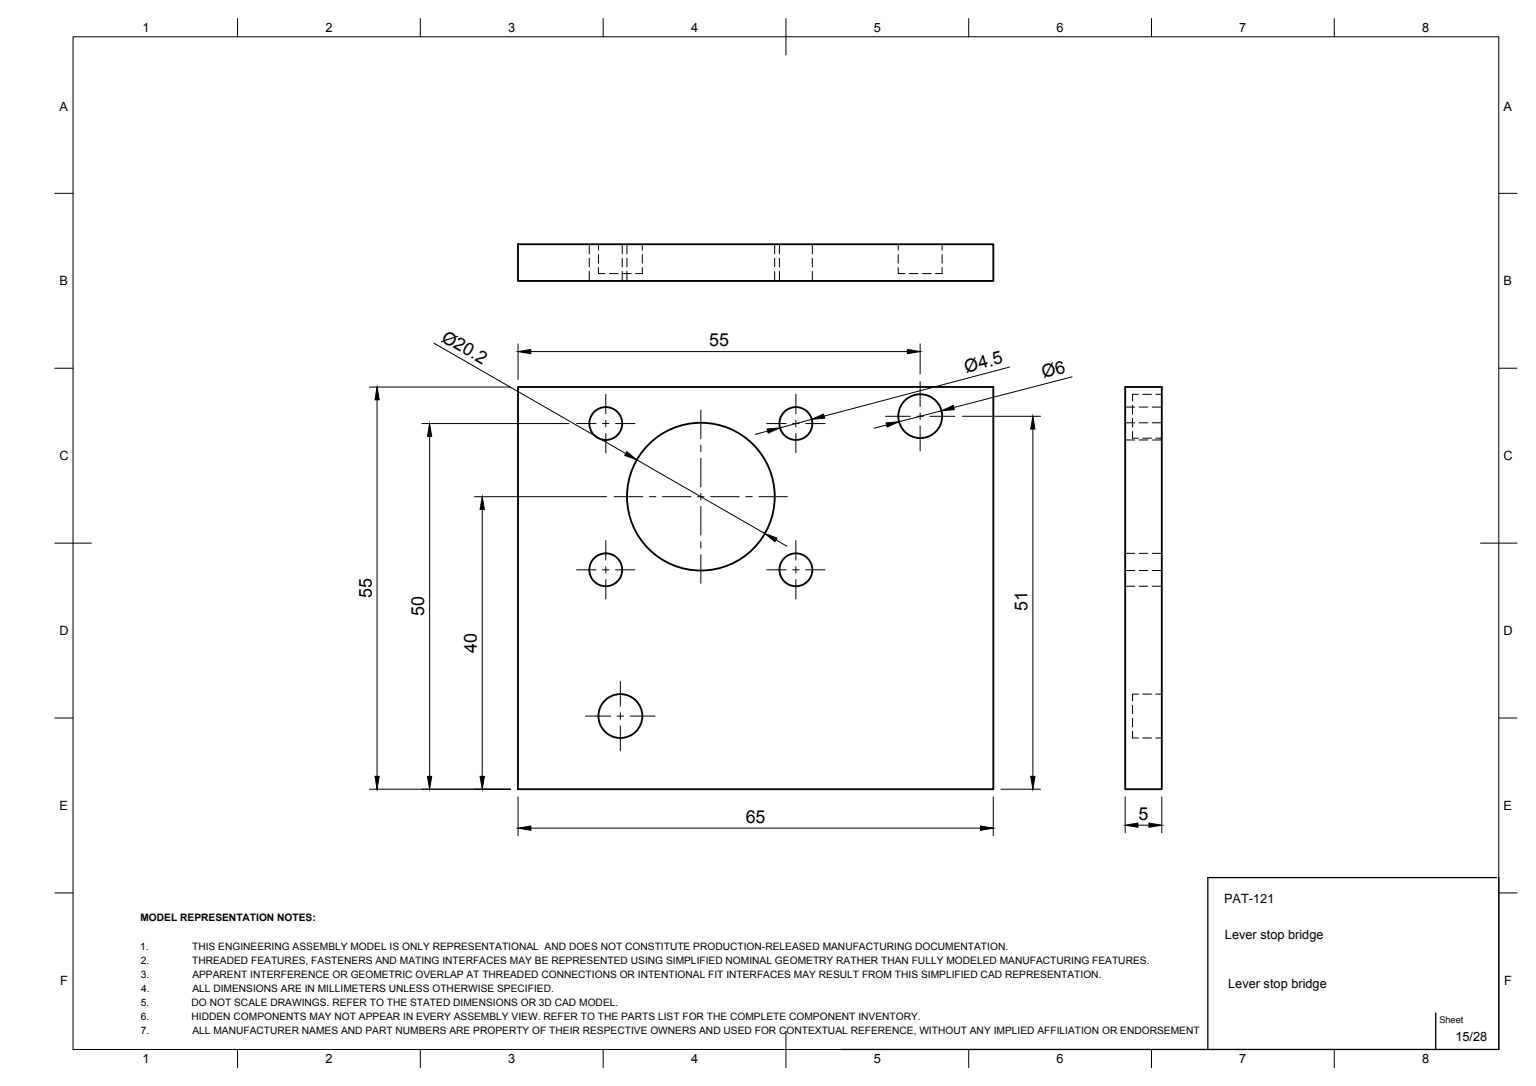
ISO-10303-21;
HEADER;
/* Generated by software containing ST-Developer
 * from STEP Tools, Inc. (www.steptools.com) 
 */

FILE_DESCRIPTION(
/* description */ ('Wall-mounted air drop station'),
/* implementation_level */ '2;1');

FILE_NAME(
/* name */ 'Lever stop bridge.step',
/* time_stamp */ '2026-10-28T22:16:19-07:00',
/* author */ (''),
/* organization */ (''),
/* preprocessor_version */ 'ST-DEVELOPER v20.2',
/* originating_system */ 'Autodesk Translation Framework v15.17.0.0',
/* authorisation */ '');

FILE_SCHEMA (('AUTOMOTIVE_DESIGN { 1 0 10303 214 3 1 1 }'));
ENDSEC;

DATA;
#10=MECHANICAL_DESIGN_GEOMETRIC_PRESENTATION_REPRESENTATION('',(#355),#10517);
#297=SHAPE_REPRESENTATION_RELATIONSHIP('SRR','None',#10654,#326);
#326=ADVANCED_BREP_SHAPE_REPRESENTATION('',(#384),#10498);
#355=STYLED_ITEM('',(#10860),#384);
#384=MANIFOLD_SOLID_BREP('Body1',#5894);
#477=FACE_BOUND('',#1356,.T.);
#478=FACE_BOUND('',#1357,.T.);
#479=FACE_BOUND('',#1358,.T.);
#480=FACE_BOUND('',#1359,.T.);
#481=FACE_BOUND('',#1360,.T.);
#482=FACE_BOUND('',#1361,.T.);
#483=FACE_BOUND('',#1362,.T.);
#484=FACE_BOUND('',#1364,.T.);
#485=FACE_BOUND('',#1365,.T.);
#486=FACE_BOUND('',#1366,.T.);
#487=FACE_BOUND('',#1367,.T.);
#488=FACE_BOUND('',#1368,.T.);
#619=PLANE('',#6528);
#620=PLANE('',#6532);
#621=PLANE('',#6548);
#622=PLANE('',#6549);
#623=PLANE('',#6550);
#624=PLANE('',#6551);
#625=PLANE('',#6552);
#626=PLANE('',#6553);
#909=FACE_OUTER_BOUND('',#1342,.T.);
#910=FACE_OUTER_BOUND('',#1343,.T.);
#911=FACE_OUTER_BOUND('',#1344,.T.);
#912=FACE_OUTER_BOUND('',#1345,.T.);
#913=FACE_OUTER_BOUND('',#1346,.T.);
#914=FACE_OUTER_BOUND('',#1347,.T.);
#915=FACE_OUTER_BOUND('',#1348,.T.);
#916=FACE_OUTER_BOUND('',#1349,.T.);
#917=FACE_OUTER_BOUND('',#1350,.T.);
#918=FACE_OUTER_BOUND('',#1351,.T.);
#919=FACE_OUTER_BOUND('',#1352,.T.);
#920=FACE_OUTER_BOUND('',#1353,.T.);
#921=FACE_OUTER_BOUND('',#1354,.T.);
#922=FACE_OUTER_BOUND('',#1355,.T.);
#923=FACE_OUTER_BOUND('',#1363,.T.);
#1342=EDGE_LOOP('',(#4631,#4632,#4633,#4634));
#1343=EDGE_LOOP('',(#4635));
#1344=EDGE_LOOP('',(#4636,#4637,#4638,#4639));
#1345=EDGE_LOOP('',(#4640));
#1346=EDGE_LOOP('',(#4641,#4642,#4643,#4644));
#1347=EDGE_LOOP('',(#4645,#4646,#4647,#4648));
#1348=EDGE_LOOP('',(#4649,#4650,#4651,#4652));
#1349=EDGE_LOOP('',(#4653,#4654,#4655,#4656));
#1350=EDGE_LOOP('',(#4657,#4658,#4659,#4660));
#1351=EDGE_LOOP('',(#4661,#4662,#4663,#4664));
#1352=EDGE_LOOP('',(#4665,#4666,#4667,#4668));
#1353=EDGE_LOOP('',(#4669,#4670,#4671,#4672));
#1354=EDGE_LOOP('',(#4673,#4674,#4675,#4676));
#1355=EDGE_LOOP('',(#4677,#4678,#4679,#4680));
#1356=EDGE_LOOP('',(#4681));
#1357=EDGE_LOOP('',(#4682));
#1358=EDGE_LOOP('',(#4683));
#1359=EDGE_LOOP('',(#4684));
#1360=EDGE_LOOP('',(#4685));
#1361=EDGE_LOOP('',(#4686));
#1362=EDGE_LOOP('',(#4687));
#1363=EDGE_LOOP('',(#4688,#4689,#4690,#4691));
#1364=EDGE_LOOP('',(#4692));
#1365=EDGE_LOOP('',(#4693));
#1366=EDGE_LOOP('',(#4694));
#1367=EDGE_LOOP('',(#4695));
#1368=EDGE_LOOP('',(#4696));
#1799=LINE('',#9486,#2263);
#1800=LINE('',#9493,#2264);
#1801=LINE('',#9500,#2265);
#1802=LINE('',#9506,#2266);
#1803=LINE('',#9512,#2267);
#1804=LINE('',#9518,#2268);
#1805=LINE('',#9524,#2269);
#1806=LINE('',#9529,#2270);
#1807=LINE('',#9531,#2271);
#1808=LINE('',#9533,#2272);
#1809=LINE('',#9534,#2273);
#1810=LINE('',#9537,#2274);
#1811=LINE('',#9539,#2275);
#1812=LINE('',#9540,#2276);
#1813=LINE('',#9543,#2277);
#1814=LINE('',#9545,#2278);
#1815=LINE('',#9546,#2279);
#1816=LINE('',#9548,#2280);
#1817=LINE('',#9549,#2281);
#2263=VECTOR('',#7715,0.3);
#2264=VECTOR('',#7724,0.3);
#2265=VECTOR('',#7733,0.225);
#2266=VECTOR('',#7740,0.225);
#2267=VECTOR('',#7747,0.225);
#2268=VECTOR('',#7754,0.225);
#2269=VECTOR('',#7761,1.01);
#2270=VECTOR('',#7766,1.);
#2271=VECTOR('',#7767,1.);
#2272=VECTOR('',#7768,1.);
#2273=VECTOR('',#7769,1.);
#2274=VECTOR('',#7772,1.);
#2275=VECTOR('',#7773,1.);
#2276=VECTOR('',#7774,1.);
#2277=VECTOR('',#7777,1.);
#2278=VECTOR('',#7778,1.);
#2279=VECTOR('',#7779,1.);
#2280=VECTOR('',#7782,1.);
#2281=VECTOR('',#7783,1.);
#2642=CIRCLE('',#6526,0.3);
#2643=CIRCLE('',#6527,0.3);
#2644=CIRCLE('',#6530,0.3);
#2645=CIRCLE('',#6531,0.3);
#2646=CIRCLE('',#6534,0.225);
#2647=CIRCLE('',#6535,0.225);
#2648=CIRCLE('',#6537,0.225);
#2649=CIRCLE('',#6538,0.225);
#2650=CIRCLE('',#6540,0.225);
#2651=CIRCLE('',#6541,0.225);
#2652=CIRCLE('',#6543,0.225);
#2653=CIRCLE('',#6544,0.225);
#2654=CIRCLE('',#6546,1.01);
#2655=CIRCLE('',#6547,1.01);
#2984=VERTEX_POINT('',#9483);
#2985=VERTEX_POINT('',#9485);
#2986=VERTEX_POINT('',#9490);
#2987=VERTEX_POINT('',#9492);
#2988=VERTEX_POINT('',#9497);
#2989=VERTEX_POINT('',#9499);
#2990=VERTEX_POINT('',#9503);
#2991=VERTEX_POINT('',#9505);
#2992=VERTEX_POINT('',#9509);
#2993=VERTEX_POINT('',#9511);
#2994=VERTEX_POINT('',#9515);
#2995=VERTEX_POINT('',#9517);
#2996=VERTEX_POINT('',#9521);
#2997=VERTEX_POINT('',#9523);
#2998=VERTEX_POINT('',#9527);
#2999=VERTEX_POINT('',#9528);
#3000=VERTEX_POINT('',#9530);
#3001=VERTEX_POINT('',#9532);
#3002=VERTEX_POINT('',#9536);
#3003=VERTEX_POINT('',#9538);
#3004=VERTEX_POINT('',#9542);
#3005=VERTEX_POINT('',#9544);
#3573=EDGE_CURVE('',#2984,#2984,#2642,.T.);
#3574=EDGE_CURVE('',#2984,#2985,#1799,.T.);
#3575=EDGE_CURVE('',#2985,#2985,#2643,.T.);
#3576=EDGE_CURVE('',#2986,#2986,#2644,.T.);
#3577=EDGE_CURVE('',#2986,#2987,#1800,.T.);
#3578=EDGE_CURVE('',#2987,#2987,#2645,.T.);
#3579=EDGE_CURVE('',#2988,#2988,#2646,.T.);
#3580=EDGE_CURVE('',#2988,#2989,#1801,.T.);
#3581=EDGE_CURVE('',#2989,#2989,#2647,.T.);
#3582=EDGE_CURVE('',#2990,#2990,#2648,.T.);
#3583=EDGE_CURVE('',#2990,#2991,#1802,.T.);
#3584=EDGE_CURVE('',#2991,#2991,#2649,.T.);
#3585=EDGE_CURVE('',#2992,#2992,#2650,.T.);
#3586=EDGE_CURVE('',#2992,#2993,#1803,.T.);
#3587=EDGE_CURVE('',#2993,#2993,#2651,.T.);
#3588=EDGE_CURVE('',#2994,#2994,#2652,.T.);
#3589=EDGE_CURVE('',#2994,#2995,#1804,.T.);
#3590=EDGE_CURVE('',#2995,#2995,#2653,.T.);
#3591=EDGE_CURVE('',#2996,#2996,#2654,.T.);
#3592=EDGE_CURVE('',#2996,#2997,#1805,.T.);
#3593=EDGE_CURVE('',#2997,#2997,#2655,.T.);
#3594=EDGE_CURVE('',#2998,#2999,#1806,.T.);
#3595=EDGE_CURVE('',#2999,#3000,#1807,.T.);
#3596=EDGE_CURVE('',#3001,#3000,#1808,.T.);
#3597=EDGE_CURVE('',#2998,#3001,#1809,.T.);
#3598=EDGE_CURVE('',#3002,#2998,#1810,.T.);
#3599=EDGE_CURVE('',#3003,#3001,#1811,.T.);
#3600=EDGE_CURVE('',#3002,#3003,#1812,.T.);
#3601=EDGE_CURVE('',#3004,#3002,#1813,.T.);
#3602=EDGE_CURVE('',#3005,#3003,#1814,.T.);
#3603=EDGE_CURVE('',#3004,#3005,#1815,.T.);
#3604=EDGE_CURVE('',#2999,#3004,#1816,.T.);
#3605=EDGE_CURVE('',#3000,#3005,#1817,.T.);
#4631=ORIENTED_EDGE('',*,*,#3573,.F.);
#4632=ORIENTED_EDGE('',*,*,#3574,.T.);
#4633=ORIENTED_EDGE('',*,*,#3575,.F.);
#4634=ORIENTED_EDGE('',*,*,#3574,.F.);
#4635=ORIENTED_EDGE('',*,*,#3573,.T.);
#4636=ORIENTED_EDGE('',*,*,#3576,.F.);
#4637=ORIENTED_EDGE('',*,*,#3577,.T.);
#4638=ORIENTED_EDGE('',*,*,#3578,.F.);
#4639=ORIENTED_EDGE('',*,*,#3577,.F.);
#4640=ORIENTED_EDGE('',*,*,#3576,.T.);
#4641=ORIENTED_EDGE('',*,*,#3579,.F.);
#4642=ORIENTED_EDGE('',*,*,#3580,.T.);
#4643=ORIENTED_EDGE('',*,*,#3581,.F.);
#4644=ORIENTED_EDGE('',*,*,#3580,.F.);
#4645=ORIENTED_EDGE('',*,*,#3582,.F.);
#4646=ORIENTED_EDGE('',*,*,#3583,.T.);
#4647=ORIENTED_EDGE('',*,*,#3584,.F.);
#4648=ORIENTED_EDGE('',*,*,#3583,.F.);
#4649=ORIENTED_EDGE('',*,*,#3585,.F.);
#4650=ORIENTED_EDGE('',*,*,#3586,.T.);
#4651=ORIENTED_EDGE('',*,*,#3587,.F.);
#4652=ORIENTED_EDGE('',*,*,#3586,.F.);
#4653=ORIENTED_EDGE('',*,*,#3588,.F.);
#4654=ORIENTED_EDGE('',*,*,#3589,.T.);
#4655=ORIENTED_EDGE('',*,*,#3590,.F.);
#4656=ORIENTED_EDGE('',*,*,#3589,.F.);
#4657=ORIENTED_EDGE('',*,*,#3591,.F.);
#4658=ORIENTED_EDGE('',*,*,#3592,.T.);
#4659=ORIENTED_EDGE('',*,*,#3593,.F.);
#4660=ORIENTED_EDGE('',*,*,#3592,.F.);
#4661=ORIENTED_EDGE('',*,*,#3594,.T.);
#4662=ORIENTED_EDGE('',*,*,#3595,.T.);
#4663=ORIENTED_EDGE('',*,*,#3596,.F.);
#4664=ORIENTED_EDGE('',*,*,#3597,.F.);
#4665=ORIENTED_EDGE('',*,*,#3598,.T.);
#4666=ORIENTED_EDGE('',*,*,#3597,.T.);
#4667=ORIENTED_EDGE('',*,*,#3599,.F.);
#4668=ORIENTED_EDGE('',*,*,#3600,.F.);
#4669=ORIENTED_EDGE('',*,*,#3601,.T.);
#4670=ORIENTED_EDGE('',*,*,#3600,.T.);
#4671=ORIENTED_EDGE('',*,*,#3602,.F.);
#4672=ORIENTED_EDGE('',*,*,#3603,.F.);
#4673=ORIENTED_EDGE('',*,*,#3604,.T.);
#4674=ORIENTED_EDGE('',*,*,#3603,.T.);
#4675=ORIENTED_EDGE('',*,*,#3605,.F.);
#4676=ORIENTED_EDGE('',*,*,#3595,.F.);
#4677=ORIENTED_EDGE('',*,*,#3605,.T.);
#4678=ORIENTED_EDGE('',*,*,#3602,.T.);
#4679=ORIENTED_EDGE('',*,*,#3599,.T.);
#4680=ORIENTED_EDGE('',*,*,#3596,.T.);
#4681=ORIENTED_EDGE('',*,*,#3575,.T.);
#4682=ORIENTED_EDGE('',*,*,#3578,.T.);
#4683=ORIENTED_EDGE('',*,*,#3593,.T.);
#4684=ORIENTED_EDGE('',*,*,#3590,.T.);
#4685=ORIENTED_EDGE('',*,*,#3587,.T.);
#4686=ORIENTED_EDGE('',*,*,#3584,.T.);
#4687=ORIENTED_EDGE('',*,*,#3581,.T.);
#4688=ORIENTED_EDGE('',*,*,#3604,.F.);
#4689=ORIENTED_EDGE('',*,*,#3594,.F.);
#4690=ORIENTED_EDGE('',*,*,#3598,.F.);
#4691=ORIENTED_EDGE('',*,*,#3601,.F.);
#4692=ORIENTED_EDGE('',*,*,#3591,.T.);
#4693=ORIENTED_EDGE('',*,*,#3588,.T.);
#4694=ORIENTED_EDGE('',*,*,#3585,.T.);
#4695=ORIENTED_EDGE('',*,*,#3582,.T.);
#4696=ORIENTED_EDGE('',*,*,#3579,.T.);
#5486=CYLINDRICAL_SURFACE('',#6525,0.3);
#5487=CYLINDRICAL_SURFACE('',#6529,0.3);
#5488=CYLINDRICAL_SURFACE('',#6533,0.225);
#5489=CYLINDRICAL_SURFACE('',#6536,0.225);
#5490=CYLINDRICAL_SURFACE('',#6539,0.225);
#5491=CYLINDRICAL_SURFACE('',#6542,0.225);
#5492=CYLINDRICAL_SURFACE('',#6545,1.01);
#5682=ADVANCED_FACE('',(#909),#5486,.F.);
#5683=ADVANCED_FACE('',(#910),#619,.T.);
#5684=ADVANCED_FACE('',(#911),#5487,.F.);
#5685=ADVANCED_FACE('',(#912),#620,.T.);
#5686=ADVANCED_FACE('',(#913),#5488,.F.);
#5687=ADVANCED_FACE('',(#914),#5489,.F.);
#5688=ADVANCED_FACE('',(#915),#5490,.F.);
#5689=ADVANCED_FACE('',(#916),#5491,.F.);
#5690=ADVANCED_FACE('',(#917),#5492,.F.);
#5691=ADVANCED_FACE('',(#918),#621,.T.);
#5692=ADVANCED_FACE('',(#919),#622,.T.);
#5693=ADVANCED_FACE('',(#920),#623,.T.);
#5694=ADVANCED_FACE('',(#921),#624,.T.);
#5695=ADVANCED_FACE('',(#922,#477,#478,#479,#480,#481,#482,#483),#625,.T.);
#5696=ADVANCED_FACE('',(#923,#484,#485,#486,#487,#488),#626,.F.);
#5894=CLOSED_SHELL('',(#5682,#5683,#5684,#5685,#5686,#5687,#5688,#5689,
#5690,#5691,#5692,#5693,#5694,#5695,#5696));
#6524=AXIS2_PLACEMENT_3D('',#9481,#7709,#7710);
#6525=AXIS2_PLACEMENT_3D('',#9482,#7711,#7712);
#6526=AXIS2_PLACEMENT_3D('',#9484,#7713,#7714);
#6527=AXIS2_PLACEMENT_3D('',#9487,#7716,#7717);
#6528=AXIS2_PLACEMENT_3D('',#9488,#7718,#7719);
#6529=AXIS2_PLACEMENT_3D('',#9489,#7720,#7721);
#6530=AXIS2_PLACEMENT_3D('',#9491,#7722,#7723);
#6531=AXIS2_PLACEMENT_3D('',#9494,#7725,#7726);
#6532=AXIS2_PLACEMENT_3D('',#9495,#7727,#7728);
#6533=AXIS2_PLACEMENT_3D('',#9496,#7729,#7730);
#6534=AXIS2_PLACEMENT_3D('',#9498,#7731,#7732);
#6535=AXIS2_PLACEMENT_3D('',#9501,#7734,#7735);
#6536=AXIS2_PLACEMENT_3D('',#9502,#7736,#7737);
#6537=AXIS2_PLACEMENT_3D('',#9504,#7738,#7739);
#6538=AXIS2_PLACEMENT_3D('',#9507,#7741,#7742);
#6539=AXIS2_PLACEMENT_3D('',#9508,#7743,#7744);
#6540=AXIS2_PLACEMENT_3D('',#9510,#7745,#7746);
#6541=AXIS2_PLACEMENT_3D('',#9513,#7748,#7749);
#6542=AXIS2_PLACEMENT_3D('',#9514,#7750,#7751);
#6543=AXIS2_PLACEMENT_3D('',#9516,#7752,#7753);
#6544=AXIS2_PLACEMENT_3D('',#9519,#7755,#7756);
#6545=AXIS2_PLACEMENT_3D('',#9520,#7757,#7758);
#6546=AXIS2_PLACEMENT_3D('',#9522,#7759,#7760);
#6547=AXIS2_PLACEMENT_3D('',#9525,#7762,#7763);
#6548=AXIS2_PLACEMENT_3D('',#9526,#7764,#7765);
#6549=AXIS2_PLACEMENT_3D('',#9535,#7770,#7771);
#6550=AXIS2_PLACEMENT_3D('',#9541,#7775,#7776);
#6551=AXIS2_PLACEMENT_3D('',#9547,#7780,#7781);
#6552=AXIS2_PLACEMENT_3D('',#9550,#7784,#7785);
#6553=AXIS2_PLACEMENT_3D('',#9551,#7786,#7787);
#7709=DIRECTION('axis',(0.,0.,1.));
#7710=DIRECTION('refdir',(1.,0.,0.));
#7711=DIRECTION('center_axis',(0.,0.,1.));
#7712=DIRECTION('ref_axis',(1.,0.,0.));
#7713=DIRECTION('center_axis',(0.,0.,1.));
#7714=DIRECTION('ref_axis',(1.,0.,0.));
#7715=DIRECTION('',(0.,0.,1.));
#7716=DIRECTION('center_axis',(0.,0.,-1.));
#7717=DIRECTION('ref_axis',(1.,0.,0.));
#7718=DIRECTION('center_axis',(0.,0.,1.));
#7719=DIRECTION('ref_axis',(1.,0.,0.));
#7720=DIRECTION('center_axis',(0.,0.,1.));
#7721=DIRECTION('ref_axis',(1.,0.,0.));
#7722=DIRECTION('center_axis',(0.,0.,1.));
#7723=DIRECTION('ref_axis',(1.,0.,0.));
#7724=DIRECTION('',(0.,0.,1.));
#7725=DIRECTION('center_axis',(0.,0.,-1.));
#7726=DIRECTION('ref_axis',(1.,0.,0.));
#7727=DIRECTION('center_axis',(0.,0.,1.));
#7728=DIRECTION('ref_axis',(1.,0.,0.));
#7729=DIRECTION('center_axis',(0.,0.,1.));
#7730=DIRECTION('ref_axis',(1.,0.,0.));
#7731=DIRECTION('center_axis',(0.,0.,1.));
#7732=DIRECTION('ref_axis',(1.,0.,0.));
#7733=DIRECTION('',(0.,0.,1.));
#7734=DIRECTION('center_axis',(0.,0.,-1.));
#7735=DIRECTION('ref_axis',(1.,0.,0.));
#7736=DIRECTION('center_axis',(0.,0.,1.));
#7737=DIRECTION('ref_axis',(1.,0.,0.));
#7738=DIRECTION('center_axis',(0.,0.,1.));
#7739=DIRECTION('ref_axis',(1.,0.,0.));
#7740=DIRECTION('',(0.,0.,1.));
#7741=DIRECTION('center_axis',(0.,0.,-1.));
#7742=DIRECTION('ref_axis',(1.,0.,0.));
#7743=DIRECTION('center_axis',(0.,0.,1.));
#7744=DIRECTION('ref_axis',(1.,0.,0.));
#7745=DIRECTION('center_axis',(0.,0.,1.));
#7746=DIRECTION('ref_axis',(1.,0.,0.));
#7747=DIRECTION('',(0.,0.,1.));
#7748=DIRECTION('center_axis',(0.,0.,-1.));
#7749=DIRECTION('ref_axis',(1.,0.,0.));
#7750=DIRECTION('center_axis',(0.,0.,1.));
#7751=DIRECTION('ref_axis',(1.,0.,0.));
#7752=DIRECTION('center_axis',(0.,0.,1.));
#7753=DIRECTION('ref_axis',(1.,0.,0.));
#7754=DIRECTION('',(0.,0.,1.));
#7755=DIRECTION('center_axis',(0.,0.,-1.));
#7756=DIRECTION('ref_axis',(1.,0.,0.));
#7757=DIRECTION('center_axis',(0.,0.,1.));
#7758=DIRECTION('ref_axis',(1.,0.,0.));
#7759=DIRECTION('center_axis',(0.,0.,1.));
#7760=DIRECTION('ref_axis',(1.,0.,0.));
#7761=DIRECTION('',(0.,0.,1.));
#7762=DIRECTION('center_axis',(0.,0.,-1.));
#7763=DIRECTION('ref_axis',(1.,0.,0.));
#7764=DIRECTION('center_axis',(0.,1.,0.));
#7765=DIRECTION('ref_axis',(-1.,0.,0.));
#7766=DIRECTION('',(-1.,0.,0.));
#7767=DIRECTION('',(0.,0.,1.));
#7768=DIRECTION('',(-1.,0.,0.));
#7769=DIRECTION('',(0.,0.,1.));
#7770=DIRECTION('center_axis',(1.,0.,0.));
#7771=DIRECTION('ref_axis',(0.,1.,0.));
#7772=DIRECTION('',(0.,1.,0.));
#7773=DIRECTION('',(0.,1.,0.));
#7774=DIRECTION('',(0.,0.,1.));
#7775=DIRECTION('center_axis',(0.,-1.,0.));
#7776=DIRECTION('ref_axis',(1.,0.,0.));
#7777=DIRECTION('',(1.,0.,0.));
#7778=DIRECTION('',(1.,0.,0.));
#7779=DIRECTION('',(0.,0.,1.));
#7780=DIRECTION('center_axis',(-1.,0.,0.));
#7781=DIRECTION('ref_axis',(0.,-1.,0.));
#7782=DIRECTION('',(0.,-1.,0.));
#7783=DIRECTION('',(0.,-1.,0.));
#7784=DIRECTION('center_axis',(0.,0.,1.));
#7785=DIRECTION('ref_axis',(1.,0.,0.));
#7786=DIRECTION('center_axis',(0.,0.,1.));
#7787=DIRECTION('ref_axis',(1.,0.,0.));
#9481=CARTESIAN_POINT('',(0.,0.,0.));
#9482=CARTESIAN_POINT('Origin',(-1.1,-3.,8.1));
#9483=CARTESIAN_POINT('',(-1.4,-3.,8.1));
#9484=CARTESIAN_POINT('Origin',(-1.1,-3.,8.1));
#9485=CARTESIAN_POINT('',(-1.4,-3.,8.5));
#9486=CARTESIAN_POINT('',(-1.4,-3.,8.1));
#9487=CARTESIAN_POINT('Origin',(-1.1,-3.,8.5));
#9488=CARTESIAN_POINT('Origin',(-1.1,-3.,8.1));
#9489=CARTESIAN_POINT('Origin',(3.,1.1,8.1));
#9490=CARTESIAN_POINT('',(2.7,1.1,8.1));
#9491=CARTESIAN_POINT('Origin',(3.,1.1,8.1));
#9492=CARTESIAN_POINT('',(2.7,1.1,8.5));
#9493=CARTESIAN_POINT('',(2.7,1.1,8.1));
#9494=CARTESIAN_POINT('Origin',(3.,1.1,8.5));
#9495=CARTESIAN_POINT('Origin',(3.,1.1,8.1));
#9496=CARTESIAN_POINT('Origin',(1.3,-1.,7.9));
#9497=CARTESIAN_POINT('',(1.075,-1.,8.));
#9498=CARTESIAN_POINT('Origin',(1.3,-1.,8.));
#9499=CARTESIAN_POINT('',(1.075,-1.,8.5));
#9500=CARTESIAN_POINT('',(1.075,-1.,7.9));
#9501=CARTESIAN_POINT('Origin',(1.3,-1.,8.5));
#9502=CARTESIAN_POINT('Origin',(-1.3,1.,7.9));
#9503=CARTESIAN_POINT('',(-1.525,1.,8.));
#9504=CARTESIAN_POINT('Origin',(-1.3,1.,8.));
#9505=CARTESIAN_POINT('',(-1.525,1.,8.5));
#9506=CARTESIAN_POINT('',(-1.525,1.,7.9));
#9507=CARTESIAN_POINT('Origin',(-1.3,1.,8.5));
#9508=CARTESIAN_POINT('Origin',(-1.3,-1.,7.9));
#9509=CARTESIAN_POINT('',(-1.525,-1.,8.));
#9510=CARTESIAN_POINT('Origin',(-1.3,-1.,8.));
#9511=CARTESIAN_POINT('',(-1.525,-1.,8.5));
#9512=CARTESIAN_POINT('',(-1.525,-1.,7.9));
#9513=CARTESIAN_POINT('Origin',(-1.3,-1.,8.5));
#9514=CARTESIAN_POINT('Origin',(1.3,1.,7.9));
#9515=CARTESIAN_POINT('',(1.075,1.,8.));
#9516=CARTESIAN_POINT('Origin',(1.3,1.,8.));
#9517=CARTESIAN_POINT('',(1.075,1.,8.5));
#9518=CARTESIAN_POINT('',(1.075,1.,7.9));
#9519=CARTESIAN_POINT('Origin',(1.3,1.,8.5));
#9520=CARTESIAN_POINT('Origin',(0.,0.,7.9));
#9521=CARTESIAN_POINT('',(-1.01,-1.23689326713883E-16,8.));
#9522=CARTESIAN_POINT('Origin',(0.,0.,8.));
#9523=CARTESIAN_POINT('',(-1.01,1.23689326713883E-16,8.5));
#9524=CARTESIAN_POINT('',(-1.01,-1.23689326713883E-16,7.9));
#9525=CARTESIAN_POINT('Origin',(0.,0.,8.5));
#9526=CARTESIAN_POINT('Origin',(4.,1.5,8.));
#9527=CARTESIAN_POINT('',(4.,1.5,8.));
#9528=CARTESIAN_POINT('',(-2.5,1.5,8.));
#9529=CARTESIAN_POINT('',(4.,1.5,8.));
#9530=CARTESIAN_POINT('',(-2.5,1.5,8.5));
#9531=CARTESIAN_POINT('',(-2.5,1.5,8.));
#9532=CARTESIAN_POINT('',(4.,1.5,8.5));
#9533=CARTESIAN_POINT('',(4.,1.5,8.5));
#9534=CARTESIAN_POINT('',(4.,1.5,8.));
#9535=CARTESIAN_POINT('Origin',(4.,-4.,8.));
#9536=CARTESIAN_POINT('',(4.,-4.,8.));
#9537=CARTESIAN_POINT('',(4.,-4.,8.));
#9538=CARTESIAN_POINT('',(4.,-4.,8.5));
#9539=CARTESIAN_POINT('',(4.,-4.,8.5));
#9540=CARTESIAN_POINT('',(4.,-4.,8.));
#9541=CARTESIAN_POINT('Origin',(-2.5,-4.,8.));
#9542=CARTESIAN_POINT('',(-2.5,-4.,8.));
#9543=CARTESIAN_POINT('',(-2.5,-4.,8.));
#9544=CARTESIAN_POINT('',(-2.5,-4.,8.5));
#9545=CARTESIAN_POINT('',(-2.5,-4.,8.5));
#9546=CARTESIAN_POINT('',(-2.5,-4.,8.));
#9547=CARTESIAN_POINT('Origin',(-2.5,1.5,8.));
#9548=CARTESIAN_POINT('',(-2.5,1.5,8.));
#9549=CARTESIAN_POINT('',(-2.5,1.5,8.5));
#9550=CARTESIAN_POINT('Origin',(0.75,-1.25,8.5));
#9551=CARTESIAN_POINT('Origin',(0.75,-1.25,8.));
#10465=UNCERTAINTY_MEASURE_WITH_UNIT(LENGTH_MEASURE(0.001),#10518,
'DISTANCE_ACCURACY_VALUE',
'Maximum model space distance between geometric entities at asserted c
onnectivities');
#10484=UNCERTAINTY_MEASURE_WITH_UNIT(LENGTH_MEASURE(0.001),#10518,
'DISTANCE_ACCURACY_VALUE',
'Maximum model space distance between geometric entities at asserted c
onnectivities');
#10498=(
GEOMETRIC_REPRESENTATION_CONTEXT(3)
GLOBAL_UNCERTAINTY_ASSIGNED_CONTEXT((#10465))
GLOBAL_UNIT_ASSIGNED_CONTEXT((#10518,#10520,#10521))
REPRESENTATION_CONTEXT('','3D')
);
#10517=(
GEOMETRIC_REPRESENTATION_CONTEXT(3)
GLOBAL_UNCERTAINTY_ASSIGNED_CONTEXT((#10484))
GLOBAL_UNIT_ASSIGNED_CONTEXT((#10518,#10520,#10521))
REPRESENTATION_CONTEXT('','3D')
);
#10518=(
LENGTH_UNIT()
NAMED_UNIT(*)
SI_UNIT(.CENTI.,.METRE.)
);
#10520=(
NAMED_UNIT(*)
PLANE_ANGLE_UNIT()
SI_UNIT($,.RADIAN.)
);
#10521=(
NAMED_UNIT(*)
SI_UNIT($,.STERADIAN.)
SOLID_ANGLE_UNIT()
);
#10535=SHAPE_DEFINITION_REPRESENTATION(#10567,#10654);
#10567=PRODUCT_DEFINITION_SHAPE('',$,#10687);
#10654=SHAPE_REPRESENTATION('',(#6524),#10498);
#10673=PRODUCT_DEFINITION_CONTEXT('part definition',#10771,'design');
#10687=PRODUCT_DEFINITION('Lever stop bridge','Lever stop bridge',#10719,
#10673);
#10719=PRODUCT_DEFINITION_FORMATION('',$,#10786);
#10771=APPLICATION_CONTEXT(
'Core Data for Automotive Mechanical Design Process');
#10772=PRODUCT_CONTEXT('part definition',#10771,'mechanical');
#10786=PRODUCT('Lever stop bridge','Lever stop bridge',
'Lever stop bridge',(#10772));
#10854=COLOUR_RGB('Light Blue',0.38,0.62,0.78);
#10855=FILL_AREA_STYLE_COLOUR('',#10854);
#10856=FILL_AREA_STYLE('',(#10855));
#10857=SURFACE_STYLE_FILL_AREA(#10856);
#10858=SURFACE_SIDE_STYLE('',(#10857));
#10859=SURFACE_STYLE_USAGE(.BOTH.,#10858);
#10860=PRESENTATION_STYLE_ASSIGNMENT((#10859));
ENDSEC;
END-ISO-10303-21;
